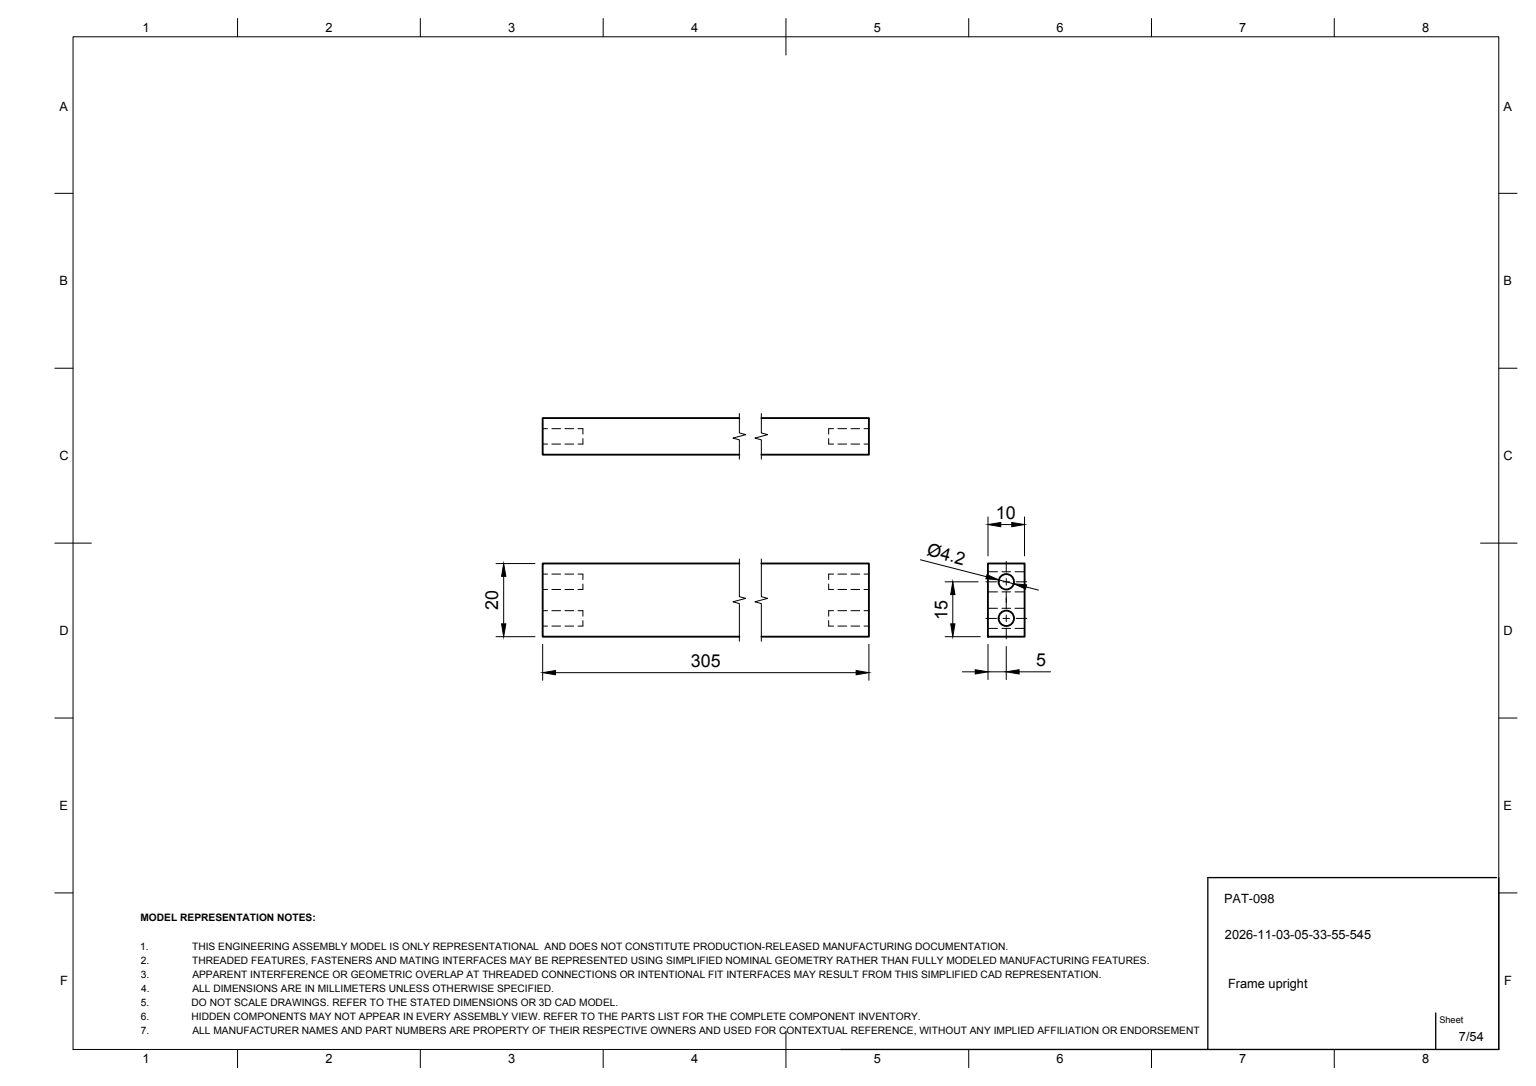
ISO-10303-21;
HEADER;
/* Generated by software containing ST-Developer
 * from STEP Tools, Inc. (www.steptools.com) 
 */

FILE_DESCRIPTION(
/* description */ ('Spring compression tester'),
/* implementation_level */ '2;1');

FILE_NAME(
/* name */ 'Frame upright.step',
/* time_stamp */ '2026-10-28T03:24:11-07:00',
/* author */ (''),
/* organization */ (''),
/* preprocessor_version */ 'ST-DEVELOPER v20.2',
/* originating_system */ 'Autodesk Translation Framework v15.17.0.0',
/* authorisation */ '');

FILE_SCHEMA (('AUTOMOTIVE_DESIGN { 1 0 10303 214 3 1 1 }'));
ENDSEC;

DATA;
#10=MECHANICAL_DESIGN_GEOMETRIC_PRESENTATION_REPRESENTATION('',(#1108),#43521);
#988=SHAPE_REPRESENTATION_RELATIONSHIP('SRR','None',#43800,#1048);
#1048=ADVANCED_BREP_SHAPE_REPRESENTATION('',(#1183),#43460);
#1108=STYLED_ITEM('',(#44181),#1183);
#1183=MANIFOLD_SOLID_BREP('Body1',#18545);
#1305=FACE_BOUND('',#3353,.T.);
#1306=FACE_BOUND('',#3354,.T.);
#1307=FACE_BOUND('',#3357,.T.);
#1308=FACE_BOUND('',#3358,.T.);
#1309=FACE_BOUND('',#3360,.T.);
#1310=FACE_BOUND('',#3361,.T.);
#1311=FACE_BOUND('',#3363,.T.);
#1312=FACE_BOUND('',#3364,.T.);
#1625=PLANE('',#19426);
#1626=PLANE('',#19430);
#1627=PLANE('',#19434);
#1628=PLANE('',#19438);
#1629=PLANE('',#19439);
#1630=PLANE('',#19440);
#1631=PLANE('',#19441);
#1632=PLANE('',#19442);
#1633=PLANE('',#19443);
#1634=PLANE('',#19444);
#2236=FACE_OUTER_BOUND('',#3341,.T.);
#2237=FACE_OUTER_BOUND('',#3342,.T.);
#2238=FACE_OUTER_BOUND('',#3343,.T.);
#2239=FACE_OUTER_BOUND('',#3344,.T.);
#2240=FACE_OUTER_BOUND('',#3345,.T.);
#2241=FACE_OUTER_BOUND('',#3346,.T.);
#2242=FACE_OUTER_BOUND('',#3347,.T.);
#2243=FACE_OUTER_BOUND('',#3348,.T.);
#2244=FACE_OUTER_BOUND('',#3349,.T.);
#2245=FACE_OUTER_BOUND('',#3350,.T.);
#2246=FACE_OUTER_BOUND('',#3351,.T.);
#2247=FACE_OUTER_BOUND('',#3352,.T.);
#2248=FACE_OUTER_BOUND('',#3355,.T.);
#2249=FACE_OUTER_BOUND('',#3356,.T.);
#2250=FACE_OUTER_BOUND('',#3359,.T.);
#2251=FACE_OUTER_BOUND('',#3362,.T.);
#3341=EDGE_LOOP('',(#12541,#12542,#12543,#12544));
#3342=EDGE_LOOP('',(#12545,#12546,#12547,#12548));
#3343=EDGE_LOOP('',(#12549,#12550,#12551,#12552));
#3344=EDGE_LOOP('',(#12553));
#3345=EDGE_LOOP('',(#12554,#12555,#12556,#12557));
#3346=EDGE_LOOP('',(#12558));
#3347=EDGE_LOOP('',(#12559,#12560,#12561,#12562));
#3348=EDGE_LOOP('',(#12563));
#3349=EDGE_LOOP('',(#12564,#12565,#12566,#12567));
#3350=EDGE_LOOP('',(#12568));
#3351=EDGE_LOOP('',(#12569,#12570,#12571,#12572));
#3352=EDGE_LOOP('',(#12573,#12574,#12575,#12576));
#3353=EDGE_LOOP('',(#12577));
#3354=EDGE_LOOP('',(#12578));
#3355=EDGE_LOOP('',(#12579,#12580,#12581,#12582));
#3356=EDGE_LOOP('',(#12583,#12584,#12585,#12586));
#3357=EDGE_LOOP('',(#12587));
#3358=EDGE_LOOP('',(#12588));
#3359=EDGE_LOOP('',(#12589,#12590,#12591,#12592));
#3360=EDGE_LOOP('',(#12593));
#3361=EDGE_LOOP('',(#12594));
#3362=EDGE_LOOP('',(#12595,#12596,#12597,#12598));
#3363=EDGE_LOOP('',(#12599));
#3364=EDGE_LOOP('',(#12600));
#4708=LINE('',#26799,#6140);
#4709=LINE('',#26805,#6141);
#4710=LINE('',#26811,#6142);
#4711=LINE('',#26818,#6143);
#4712=LINE('',#26825,#6144);
#4713=LINE('',#26832,#6145);
#4714=LINE('',#26838,#6146);
#4715=LINE('',#26840,#6147);
#4716=LINE('',#26842,#6148);
#4717=LINE('',#26843,#6149);
#4718=LINE('',#26846,#6150);
#4719=LINE('',#26848,#6151);
#4720=LINE('',#26849,#6152);
#4721=LINE('',#26852,#6153);
#4722=LINE('',#26854,#6154);
#4723=LINE('',#26855,#6155);
#4724=LINE('',#26857,#6156);
#4725=LINE('',#26858,#6157);
#6140=VECTOR('',#21568,0.274999999999999);
#6141=VECTOR('',#21575,0.274999999999999);
#6142=VECTOR('',#21582,0.21);
#6143=VECTOR('',#21591,0.21);
#6144=VECTOR('',#21600,0.21);
#6145=VECTOR('',#21609,0.21);
#6146=VECTOR('',#21616,1.);
#6147=VECTOR('',#21617,1.);
#6148=VECTOR('',#21618,1.);
#6149=VECTOR('',#21619,1.);
#6150=VECTOR('',#21622,1.);
#6151=VECTOR('',#21623,1.);
#6152=VECTOR('',#21624,1.);
#6153=VECTOR('',#21627,1.);
#6154=VECTOR('',#21628,1.);
#6155=VECTOR('',#21629,1.);
#6156=VECTOR('',#21632,1.);
#6157=VECTOR('',#21633,1.);
#7530=CIRCLE('',#19418,0.274999999999999);
#7531=CIRCLE('',#19419,0.274999999999999);
#7532=CIRCLE('',#19421,0.274999999999999);
#7533=CIRCLE('',#19422,0.274999999999999);
#7534=CIRCLE('',#19424,0.21);
#7535=CIRCLE('',#19425,0.21);
#7536=CIRCLE('',#19428,0.21);
#7537=CIRCLE('',#19429,0.21);
#7538=CIRCLE('',#19432,0.21);
#7539=CIRCLE('',#19433,0.21);
#7540=CIRCLE('',#19436,0.21);
#7541=CIRCLE('',#19437,0.21);
#8244=VERTEX_POINT('',#26796);
#8245=VERTEX_POINT('',#26798);
#8246=VERTEX_POINT('',#26802);
#8247=VERTEX_POINT('',#26804);
#8248=VERTEX_POINT('',#26808);
#8249=VERTEX_POINT('',#26810);
#8250=VERTEX_POINT('',#26815);
#8251=VERTEX_POINT('',#26817);
#8252=VERTEX_POINT('',#26822);
#8253=VERTEX_POINT('',#26824);
#8254=VERTEX_POINT('',#26829);
#8255=VERTEX_POINT('',#26831);
#8256=VERTEX_POINT('',#26836);
#8257=VERTEX_POINT('',#26837);
#8258=VERTEX_POINT('',#26839);
#8259=VERTEX_POINT('',#26841);
#8260=VERTEX_POINT('',#26845);
#8261=VERTEX_POINT('',#26847);
#8262=VERTEX_POINT('',#26851);
#8263=VERTEX_POINT('',#26853);
#9935=EDGE_CURVE('',#8244,#8244,#7530,.T.);
#9936=EDGE_CURVE('',#8244,#8245,#4708,.T.);
#9937=EDGE_CURVE('',#8245,#8245,#7531,.T.);
#9938=EDGE_CURVE('',#8246,#8246,#7532,.T.);
#9939=EDGE_CURVE('',#8246,#8247,#4709,.T.);
#9940=EDGE_CURVE('',#8247,#8247,#7533,.T.);
#9941=EDGE_CURVE('',#8248,#8248,#7534,.T.);
#9942=EDGE_CURVE('',#8248,#8249,#4710,.T.);
#9943=EDGE_CURVE('',#8249,#8249,#7535,.T.);
#9944=EDGE_CURVE('',#8250,#8250,#7536,.T.);
#9945=EDGE_CURVE('',#8250,#8251,#4711,.T.);
#9946=EDGE_CURVE('',#8251,#8251,#7537,.T.);
#9947=EDGE_CURVE('',#8252,#8252,#7538,.T.);
#9948=EDGE_CURVE('',#8252,#8253,#4712,.T.);
#9949=EDGE_CURVE('',#8253,#8253,#7539,.T.);
#9950=EDGE_CURVE('',#8254,#8254,#7540,.T.);
#9951=EDGE_CURVE('',#8254,#8255,#4713,.T.);
#9952=EDGE_CURVE('',#8255,#8255,#7541,.T.);
#9953=EDGE_CURVE('',#8256,#8257,#4714,.T.);
#9954=EDGE_CURVE('',#8257,#8258,#4715,.T.);
#9955=EDGE_CURVE('',#8259,#8258,#4716,.T.);
#9956=EDGE_CURVE('',#8256,#8259,#4717,.T.);
#9957=EDGE_CURVE('',#8260,#8256,#4718,.T.);
#9958=EDGE_CURVE('',#8261,#8259,#4719,.T.);
#9959=EDGE_CURVE('',#8260,#8261,#4720,.T.);
#9960=EDGE_CURVE('',#8262,#8260,#4721,.T.);
#9961=EDGE_CURVE('',#8263,#8261,#4722,.T.);
#9962=EDGE_CURVE('',#8262,#8263,#4723,.T.);
#9963=EDGE_CURVE('',#8257,#8262,#4724,.T.);
#9964=EDGE_CURVE('',#8258,#8263,#4725,.T.);
#12541=ORIENTED_EDGE('',*,*,#9935,.F.);
#12542=ORIENTED_EDGE('',*,*,#9936,.T.);
#12543=ORIENTED_EDGE('',*,*,#9937,.F.);
#12544=ORIENTED_EDGE('',*,*,#9936,.F.);
#12545=ORIENTED_EDGE('',*,*,#9938,.F.);
#12546=ORIENTED_EDGE('',*,*,#9939,.T.);
#12547=ORIENTED_EDGE('',*,*,#9940,.F.);
#12548=ORIENTED_EDGE('',*,*,#9939,.F.);
#12549=ORIENTED_EDGE('',*,*,#9941,.F.);
#12550=ORIENTED_EDGE('',*,*,#9942,.T.);
#12551=ORIENTED_EDGE('',*,*,#9943,.F.);
#12552=ORIENTED_EDGE('',*,*,#9942,.F.);
#12553=ORIENTED_EDGE('',*,*,#9941,.T.);
#12554=ORIENTED_EDGE('',*,*,#9944,.F.);
#12555=ORIENTED_EDGE('',*,*,#9945,.T.);
#12556=ORIENTED_EDGE('',*,*,#9946,.F.);
#12557=ORIENTED_EDGE('',*,*,#9945,.F.);
#12558=ORIENTED_EDGE('',*,*,#9944,.T.);
#12559=ORIENTED_EDGE('',*,*,#9947,.F.);
#12560=ORIENTED_EDGE('',*,*,#9948,.T.);
#12561=ORIENTED_EDGE('',*,*,#9949,.T.);
#12562=ORIENTED_EDGE('',*,*,#9948,.F.);
#12563=ORIENTED_EDGE('',*,*,#9949,.F.);
#12564=ORIENTED_EDGE('',*,*,#9950,.F.);
#12565=ORIENTED_EDGE('',*,*,#9951,.T.);
#12566=ORIENTED_EDGE('',*,*,#9952,.T.);
#12567=ORIENTED_EDGE('',*,*,#9951,.F.);
#12568=ORIENTED_EDGE('',*,*,#9952,.F.);
#12569=ORIENTED_EDGE('',*,*,#9953,.T.);
#12570=ORIENTED_EDGE('',*,*,#9954,.T.);
#12571=ORIENTED_EDGE('',*,*,#9955,.F.);
#12572=ORIENTED_EDGE('',*,*,#9956,.F.);
#12573=ORIENTED_EDGE('',*,*,#9957,.T.);
#12574=ORIENTED_EDGE('',*,*,#9956,.T.);
#12575=ORIENTED_EDGE('',*,*,#9958,.F.);
#12576=ORIENTED_EDGE('',*,*,#9959,.F.);
#12577=ORIENTED_EDGE('',*,*,#9937,.T.);
#12578=ORIENTED_EDGE('',*,*,#9940,.T.);
#12579=ORIENTED_EDGE('',*,*,#9960,.T.);
#12580=ORIENTED_EDGE('',*,*,#9959,.T.);
#12581=ORIENTED_EDGE('',*,*,#9961,.F.);
#12582=ORIENTED_EDGE('',*,*,#9962,.F.);
#12583=ORIENTED_EDGE('',*,*,#9963,.T.);
#12584=ORIENTED_EDGE('',*,*,#9962,.T.);
#12585=ORIENTED_EDGE('',*,*,#9964,.F.);
#12586=ORIENTED_EDGE('',*,*,#9954,.F.);
#12587=ORIENTED_EDGE('',*,*,#9935,.T.);
#12588=ORIENTED_EDGE('',*,*,#9938,.T.);
#12589=ORIENTED_EDGE('',*,*,#9964,.T.);
#12590=ORIENTED_EDGE('',*,*,#9961,.T.);
#12591=ORIENTED_EDGE('',*,*,#9958,.T.);
#12592=ORIENTED_EDGE('',*,*,#9955,.T.);
#12593=ORIENTED_EDGE('',*,*,#9943,.T.);
#12594=ORIENTED_EDGE('',*,*,#9946,.T.);
#12595=ORIENTED_EDGE('',*,*,#9963,.F.);
#12596=ORIENTED_EDGE('',*,*,#9953,.F.);
#12597=ORIENTED_EDGE('',*,*,#9957,.F.);
#12598=ORIENTED_EDGE('',*,*,#9960,.F.);
#12599=ORIENTED_EDGE('',*,*,#9947,.T.);
#12600=ORIENTED_EDGE('',*,*,#9950,.T.);
#17135=CYLINDRICAL_SURFACE('',#19417,0.274999999999999);
#17136=CYLINDRICAL_SURFACE('',#19420,0.274999999999999);
#17137=CYLINDRICAL_SURFACE('',#19423,0.21);
#17138=CYLINDRICAL_SURFACE('',#19427,0.21);
#17139=CYLINDRICAL_SURFACE('',#19431,0.21);
#17140=CYLINDRICAL_SURFACE('',#19435,0.21);
#17560=ADVANCED_FACE('',(#2236),#17135,.F.);
#17561=ADVANCED_FACE('',(#2237),#17136,.F.);
#17562=ADVANCED_FACE('',(#2238),#17137,.F.);
#17563=ADVANCED_FACE('',(#2239),#1625,.T.);
#17564=ADVANCED_FACE('',(#2240),#17138,.F.);
#17565=ADVANCED_FACE('',(#2241),#1626,.T.);
#17566=ADVANCED_FACE('',(#2242),#17139,.F.);
#17567=ADVANCED_FACE('',(#2243),#1627,.F.);
#17568=ADVANCED_FACE('',(#2244),#17140,.F.);
#17569=ADVANCED_FACE('',(#2245),#1628,.F.);
#17570=ADVANCED_FACE('',(#2246),#1629,.T.);
#17571=ADVANCED_FACE('',(#2247,#1305,#1306),#1630,.T.);
#17572=ADVANCED_FACE('',(#2248),#1631,.T.);
#17573=ADVANCED_FACE('',(#2249,#1307,#1308),#1632,.T.);
#17574=ADVANCED_FACE('',(#2250,#1309,#1310),#1633,.T.);
#17575=ADVANCED_FACE('',(#2251,#1311,#1312),#1634,.F.);
#18545=CLOSED_SHELL('',(#17560,#17561,#17562,#17563,#17564,#17565,#17566,
#17567,#17568,#17569,#17570,#17571,#17572,#17573,#17574,#17575));
#19416=AXIS2_PLACEMENT_3D('',#26794,#21562,#21563);
#19417=AXIS2_PLACEMENT_3D('',#26795,#21564,#21565);
#19418=AXIS2_PLACEMENT_3D('',#26797,#21566,#21567);
#19419=AXIS2_PLACEMENT_3D('',#26800,#21569,#21570);
#19420=AXIS2_PLACEMENT_3D('',#26801,#21571,#21572);
#19421=AXIS2_PLACEMENT_3D('',#26803,#21573,#21574);
#19422=AXIS2_PLACEMENT_3D('',#26806,#21576,#21577);
#19423=AXIS2_PLACEMENT_3D('',#26807,#21578,#21579);
#19424=AXIS2_PLACEMENT_3D('',#26809,#21580,#21581);
#19425=AXIS2_PLACEMENT_3D('',#26812,#21583,#21584);
#19426=AXIS2_PLACEMENT_3D('',#26813,#21585,#21586);
#19427=AXIS2_PLACEMENT_3D('',#26814,#21587,#21588);
#19428=AXIS2_PLACEMENT_3D('',#26816,#21589,#21590);
#19429=AXIS2_PLACEMENT_3D('',#26819,#21592,#21593);
#19430=AXIS2_PLACEMENT_3D('',#26820,#21594,#21595);
#19431=AXIS2_PLACEMENT_3D('',#26821,#21596,#21597);
#19432=AXIS2_PLACEMENT_3D('',#26823,#21598,#21599);
#19433=AXIS2_PLACEMENT_3D('',#26826,#21601,#21602);
#19434=AXIS2_PLACEMENT_3D('',#26827,#21603,#21604);
#19435=AXIS2_PLACEMENT_3D('',#26828,#21605,#21606);
#19436=AXIS2_PLACEMENT_3D('',#26830,#21607,#21608);
#19437=AXIS2_PLACEMENT_3D('',#26833,#21610,#21611);
#19438=AXIS2_PLACEMENT_3D('',#26834,#21612,#21613);
#19439=AXIS2_PLACEMENT_3D('',#26835,#21614,#21615);
#19440=AXIS2_PLACEMENT_3D('',#26844,#21620,#21621);
#19441=AXIS2_PLACEMENT_3D('',#26850,#21625,#21626);
#19442=AXIS2_PLACEMENT_3D('',#26856,#21630,#21631);
#19443=AXIS2_PLACEMENT_3D('',#26859,#21634,#21635);
#19444=AXIS2_PLACEMENT_3D('',#26860,#21636,#21637);
#21562=DIRECTION('axis',(0.,0.,1.));
#21563=DIRECTION('refdir',(1.,0.,0.));
#21564=DIRECTION('center_axis',(1.,0.,0.));
#21565=DIRECTION('ref_axis',(0.,0.,-1.));
#21566=DIRECTION('center_axis',(1.,0.,0.));
#21567=DIRECTION('ref_axis',(0.,0.,-1.));
#21568=DIRECTION('',(1.,0.,0.));
#21569=DIRECTION('center_axis',(-1.,0.,0.));
#21570=DIRECTION('ref_axis',(0.,0.,-1.));
#21571=DIRECTION('center_axis',(1.,0.,0.));
#21572=DIRECTION('ref_axis',(0.,0.,-1.));
#21573=DIRECTION('center_axis',(1.,0.,0.));
#21574=DIRECTION('ref_axis',(0.,0.,-1.));
#21575=DIRECTION('',(1.,0.,0.));
#21576=DIRECTION('center_axis',(-1.,0.,0.));
#21577=DIRECTION('ref_axis',(0.,0.,-1.));
#21578=DIRECTION('center_axis',(0.,0.,1.));
#21579=DIRECTION('ref_axis',(1.,0.,0.));
#21580=DIRECTION('center_axis',(0.,0.,1.));
#21581=DIRECTION('ref_axis',(1.,0.,0.));
#21582=DIRECTION('',(0.,0.,1.));
#21583=DIRECTION('center_axis',(0.,0.,-1.));
#21584=DIRECTION('ref_axis',(1.,0.,0.));
#21585=DIRECTION('center_axis',(0.,0.,1.));
#21586=DIRECTION('ref_axis',(1.,0.,0.));
#21587=DIRECTION('center_axis',(0.,0.,1.));
#21588=DIRECTION('ref_axis',(1.,0.,0.));
#21589=DIRECTION('center_axis',(0.,0.,1.));
#21590=DIRECTION('ref_axis',(1.,0.,0.));
#21591=DIRECTION('',(0.,0.,1.));
#21592=DIRECTION('center_axis',(0.,0.,-1.));
#21593=DIRECTION('ref_axis',(1.,0.,0.));
#21594=DIRECTION('center_axis',(0.,0.,1.));
#21595=DIRECTION('ref_axis',(1.,0.,0.));
#21596=DIRECTION('center_axis',(0.,0.,1.));
#21597=DIRECTION('ref_axis',(1.,0.,0.));
#21598=DIRECTION('center_axis',(0.,0.,1.));
#21599=DIRECTION('ref_axis',(1.,0.,0.));
#21600=DIRECTION('',(0.,0.,1.));
#21601=DIRECTION('center_axis',(0.,0.,1.));
#21602=DIRECTION('ref_axis',(1.,0.,0.));
#21603=DIRECTION('center_axis',(0.,0.,1.));
#21604=DIRECTION('ref_axis',(1.,0.,0.));
#21605=DIRECTION('center_axis',(0.,0.,1.));
#21606=DIRECTION('ref_axis',(1.,0.,0.));
#21607=DIRECTION('center_axis',(0.,0.,1.));
#21608=DIRECTION('ref_axis',(1.,0.,0.));
#21609=DIRECTION('',(0.,0.,1.));
#21610=DIRECTION('center_axis',(0.,0.,1.));
#21611=DIRECTION('ref_axis',(1.,0.,0.));
#21612=DIRECTION('center_axis',(0.,0.,1.));
#21613=DIRECTION('ref_axis',(1.,0.,0.));
#21614=DIRECTION('center_axis',(0.,1.,0.));
#21615=DIRECTION('ref_axis',(-1.,0.,0.));
#21616=DIRECTION('',(-1.,0.,0.));
#21617=DIRECTION('',(0.,0.,1.));
#21618=DIRECTION('',(-1.,0.,0.));
#21619=DIRECTION('',(0.,0.,1.));
#21620=DIRECTION('center_axis',(1.,0.,0.));
#21621=DIRECTION('ref_axis',(0.,1.,0.));
#21622=DIRECTION('',(0.,1.,0.));
#21623=DIRECTION('',(0.,1.,0.));
#21624=DIRECTION('',(0.,0.,1.));
#21625=DIRECTION('center_axis',(0.,-1.,0.));
#21626=DIRECTION('ref_axis',(1.,0.,0.));
#21627=DIRECTION('',(1.,0.,0.));
#21628=DIRECTION('',(1.,0.,0.));
#21629=DIRECTION('',(0.,0.,1.));
#21630=DIRECTION('center_axis',(-1.,0.,0.));
#21631=DIRECTION('ref_axis',(0.,-1.,0.));
#21632=DIRECTION('',(0.,-1.,0.));
#21633=DIRECTION('',(0.,-1.,0.));
#21634=DIRECTION('center_axis',(0.,0.,1.));
#21635=DIRECTION('ref_axis',(1.,0.,0.));
#21636=DIRECTION('center_axis',(0.,0.,1.));
#21637=DIRECTION('ref_axis',(1.,0.,0.));
#26794=CARTESIAN_POINT('',(0.,0.,0.));
#26795=CARTESIAN_POINT('Origin',(-7.6,9.5,24.));
#26796=CARTESIAN_POINT('',(-7.5,9.5,24.275));
#26797=CARTESIAN_POINT('Origin',(-7.5,9.5,24.));
#26798=CARTESIAN_POINT('',(-6.5,9.5,24.275));
#26799=CARTESIAN_POINT('',(-7.6,9.5,24.275));
#26800=CARTESIAN_POINT('Origin',(-6.5,9.5,24.));
#26801=CARTESIAN_POINT('Origin',(-7.6,10.5,24.));
#26802=CARTESIAN_POINT('',(-7.5,10.5,24.275));
#26803=CARTESIAN_POINT('Origin',(-7.5,10.5,24.));
#26804=CARTESIAN_POINT('',(-6.5,10.5,24.275));
#26805=CARTESIAN_POINT('',(-7.6,10.5,24.275));
#26806=CARTESIAN_POINT('Origin',(-6.5,10.5,24.));
#26807=CARTESIAN_POINT('Origin',(-7.,9.5,29.4));
#26808=CARTESIAN_POINT('',(-7.21,9.5,29.4));
#26809=CARTESIAN_POINT('Origin',(-7.,9.5,29.4));
#26810=CARTESIAN_POINT('',(-7.21,9.5,30.5));
#26811=CARTESIAN_POINT('',(-7.21,9.5,29.4));
#26812=CARTESIAN_POINT('Origin',(-7.,9.5,30.5));
#26813=CARTESIAN_POINT('Origin',(-7.,9.5,29.4));
#26814=CARTESIAN_POINT('Origin',(-7.,10.5,29.4));
#26815=CARTESIAN_POINT('',(-7.21,10.5,29.4));
#26816=CARTESIAN_POINT('Origin',(-7.,10.5,29.4));
#26817=CARTESIAN_POINT('',(-7.21,10.5,30.5));
#26818=CARTESIAN_POINT('',(-7.21,10.5,29.4));
#26819=CARTESIAN_POINT('Origin',(-7.,10.5,30.5));
#26820=CARTESIAN_POINT('Origin',(-7.,10.5,29.4));
#26821=CARTESIAN_POINT('Origin',(-7.,9.5,-0.1));
#26822=CARTESIAN_POINT('',(-7.21,9.5,0.));
#26823=CARTESIAN_POINT('Origin',(-7.,9.5,0.));
#26824=CARTESIAN_POINT('',(-7.21,9.5,1.1));
#26825=CARTESIAN_POINT('',(-7.21,9.5,-0.1));
#26826=CARTESIAN_POINT('Origin',(-7.,9.5,1.1));
#26827=CARTESIAN_POINT('Origin',(-7.,9.5,1.1));
#26828=CARTESIAN_POINT('Origin',(-7.,10.5,-0.1));
#26829=CARTESIAN_POINT('',(-7.21,10.5,0.));
#26830=CARTESIAN_POINT('Origin',(-7.,10.5,0.));
#26831=CARTESIAN_POINT('',(-7.21,10.5,1.1));
#26832=CARTESIAN_POINT('',(-7.21,10.5,-0.1));
#26833=CARTESIAN_POINT('Origin',(-7.,10.5,1.1));
#26834=CARTESIAN_POINT('Origin',(-7.,10.5,1.1));
#26835=CARTESIAN_POINT('Origin',(-6.5,11.,0.));
#26836=CARTESIAN_POINT('',(-6.5,11.,0.));
#26837=CARTESIAN_POINT('',(-7.5,11.,0.));
#26838=CARTESIAN_POINT('',(-6.5,11.,0.));
#26839=CARTESIAN_POINT('',(-7.5,11.,30.5));
#26840=CARTESIAN_POINT('',(-7.5,11.,0.));
#26841=CARTESIAN_POINT('',(-6.5,11.,30.5));
#26842=CARTESIAN_POINT('',(-6.5,11.,30.5));
#26843=CARTESIAN_POINT('',(-6.5,11.,0.));
#26844=CARTESIAN_POINT('Origin',(-6.5,9.,0.));
#26845=CARTESIAN_POINT('',(-6.5,9.,0.));
#26846=CARTESIAN_POINT('',(-6.5,9.,0.));
#26847=CARTESIAN_POINT('',(-6.5,9.,30.5));
#26848=CARTESIAN_POINT('',(-6.5,9.,30.5));
#26849=CARTESIAN_POINT('',(-6.5,9.,0.));
#26850=CARTESIAN_POINT('Origin',(-7.5,9.,0.));
#26851=CARTESIAN_POINT('',(-7.5,9.,0.));
#26852=CARTESIAN_POINT('',(-7.5,9.,0.));
#26853=CARTESIAN_POINT('',(-7.5,9.,30.5));
#26854=CARTESIAN_POINT('',(-7.5,9.,30.5));
#26855=CARTESIAN_POINT('',(-7.5,9.,0.));
#26856=CARTESIAN_POINT('Origin',(-7.5,11.,0.));
#26857=CARTESIAN_POINT('',(-7.5,11.,0.));
#26858=CARTESIAN_POINT('',(-7.5,11.,30.5));
#26859=CARTESIAN_POINT('Origin',(-7.,10.,30.5));
#26860=CARTESIAN_POINT('Origin',(-7.,10.,0.));
#43392=UNCERTAINTY_MEASURE_WITH_UNIT(LENGTH_MEASURE(0.001),#43522,
'DISTANCE_ACCURACY_VALUE',
'Maximum model space distance between geometric entities at asserted c
onnectivities');
#43453=UNCERTAINTY_MEASURE_WITH_UNIT(LENGTH_MEASURE(0.001),#43522,
'DISTANCE_ACCURACY_VALUE',
'Maximum model space distance between geometric entities at asserted c
onnectivities');
#43460=(
GEOMETRIC_REPRESENTATION_CONTEXT(3)
GLOBAL_UNCERTAINTY_ASSIGNED_CONTEXT((#43392))
GLOBAL_UNIT_ASSIGNED_CONTEXT((#43522,#43524,#43525))
REPRESENTATION_CONTEXT('','3D')
);
#43521=(
GEOMETRIC_REPRESENTATION_CONTEXT(3)
GLOBAL_UNCERTAINTY_ASSIGNED_CONTEXT((#43453))
GLOBAL_UNIT_ASSIGNED_CONTEXT((#43522,#43524,#43525))
REPRESENTATION_CONTEXT('','3D')
);
#43522=(
LENGTH_UNIT()
NAMED_UNIT(*)
SI_UNIT(.CENTI.,.METRE.)
);
#43524=(
NAMED_UNIT(*)
PLANE_ANGLE_UNIT()
SI_UNIT($,.RADIAN.)
);
#43525=(
NAMED_UNIT(*)
SI_UNIT($,.STERADIAN.)
SOLID_ANGLE_UNIT()
);
#43532=SHAPE_DEFINITION_REPRESENTATION(#43599,#43800);
#43599=PRODUCT_DEFINITION_SHAPE('',$,#43868);
#43800=SHAPE_REPRESENTATION('',(#19416),#43460);
#43861=PRODUCT_DEFINITION_CONTEXT('part definition',#44064,'design');
#43868=PRODUCT_DEFINITION('Frame upright','Frame upright',#43935,#43861);
#43935=PRODUCT_DEFINITION_FORMATION('',$,#44072);
#44064=APPLICATION_CONTEXT(
'Core Data for Automotive Mechanical Design Process');
#44065=PRODUCT_CONTEXT('part definition',#44064,'mechanical');
#44072=PRODUCT('Frame upright','Frame upright','Frame upright',(#44065));
#44175=COLOUR_RGB('Dark Blue',0.08,0.2,0.34);
#44176=FILL_AREA_STYLE_COLOUR('',#44175);
#44177=FILL_AREA_STYLE('',(#44176));
#44178=SURFACE_STYLE_FILL_AREA(#44177);
#44179=SURFACE_SIDE_STYLE('',(#44178));
#44180=SURFACE_STYLE_USAGE(.BOTH.,#44179);
#44181=PRESENTATION_STYLE_ASSIGNMENT((#44180));
ENDSEC;
END-ISO-10303-21;
